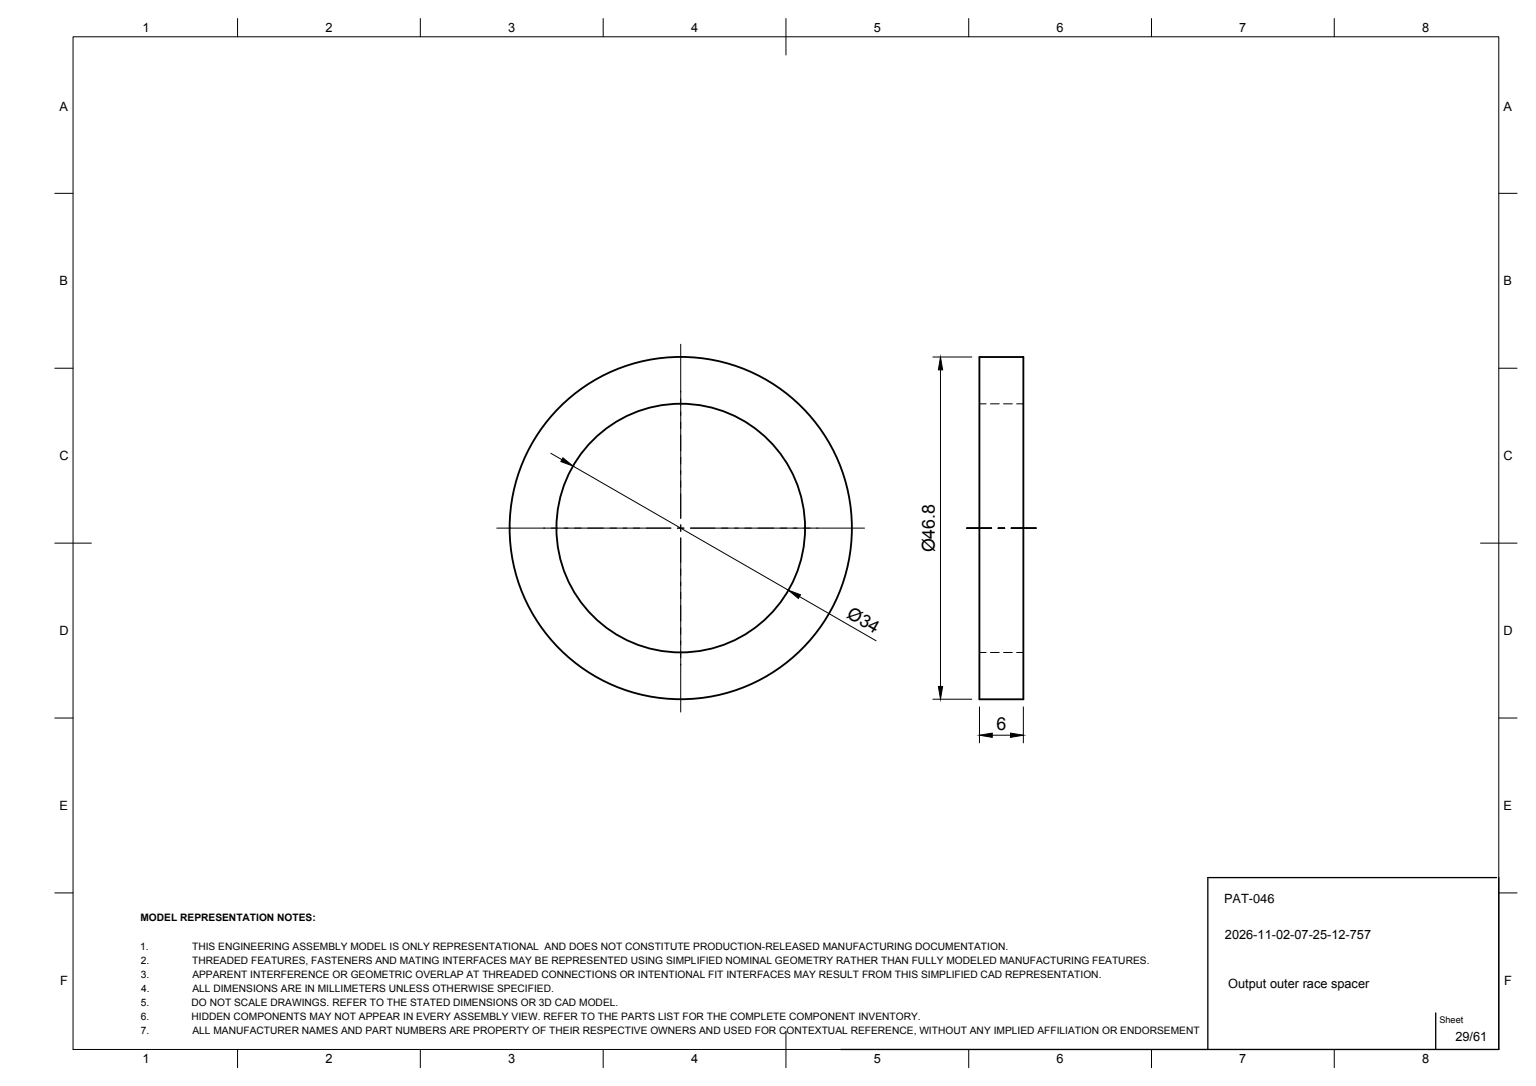
ISO-10303-21;
HEADER;
/* Generated by software containing ST-Developer
 * from STEP Tools, Inc. (www.steptools.com) 
 */

FILE_DESCRIPTION(
/* description */ ('Gear mesh backlash fixture'),
/* implementation_level */ '2;1');

FILE_NAME(
/* name */ 'Output outer race spacer.step',
/* time_stamp */ '2026-10-28T03:26:00-07:00',
/* author */ (''),
/* organization */ (''),
/* preprocessor_version */ 'ST-DEVELOPER v20.2',
/* originating_system */ 'Autodesk Translation Framework v15.17.0.0',
/* authorisation */ '');

FILE_SCHEMA (('AUTOMOTIVE_DESIGN { 1 0 10303 214 3 1 1 }'));
ENDSEC;

DATA;
#10=MECHANICAL_DESIGN_GEOMETRIC_PRESENTATION_REPRESENTATION('',(#1044),#57900);
#937=SHAPE_REPRESENTATION_RELATIONSHIP('SRR','None',#58134,#987);
#987=ADVANCED_BREP_SHAPE_REPRESENTATION('',(#1108),#57867);
#1044=STYLED_ITEM('',(#58465),#1108);
#1108=MANIFOLD_SOLID_BREP('Body1',#13605);
#1264=FACE_BOUND('',#2851,.T.);
#1265=FACE_BOUND('',#2853,.T.);
#1470=PLANE('',#14778);
#1471=PLANE('',#14779);
#1962=FACE_OUTER_BOUND('',#2848,.T.);
#1963=FACE_OUTER_BOUND('',#2849,.T.);
#1964=FACE_OUTER_BOUND('',#2850,.T.);
#1965=FACE_OUTER_BOUND('',#2852,.T.);
#2848=EDGE_LOOP('',(#10077,#10078,#10079,#10080));
#2849=EDGE_LOOP('',(#10081,#10082,#10083,#10084));
#2850=EDGE_LOOP('',(#10085));
#2851=EDGE_LOOP('',(#10086));
#2852=EDGE_LOOP('',(#10087));
#2853=EDGE_LOOP('',(#10088));
#3707=LINE('',#20994,#4596);
#3708=LINE('',#21000,#4597);
#4596=VECTOR('',#17032,1.7);
#4597=VECTOR('',#17039,2.34);
#5467=CIRCLE('',#14773,1.7);
#5468=CIRCLE('',#14774,1.7);
#5469=CIRCLE('',#14776,2.34);
#5470=CIRCLE('',#14777,2.34);
#6183=VERTEX_POINT('',#20991);
#6184=VERTEX_POINT('',#20993);
#6185=VERTEX_POINT('',#20997);
#6186=VERTEX_POINT('',#20999);
#7625=EDGE_CURVE('',#6183,#6183,#5467,.T.);
#7626=EDGE_CURVE('',#6183,#6184,#3707,.T.);
#7627=EDGE_CURVE('',#6184,#6184,#5468,.T.);
#7628=EDGE_CURVE('',#6185,#6185,#5469,.T.);
#7629=EDGE_CURVE('',#6185,#6186,#3708,.T.);
#7630=EDGE_CURVE('',#6186,#6186,#5470,.T.);
#10077=ORIENTED_EDGE('',*,*,#7625,.F.);
#10078=ORIENTED_EDGE('',*,*,#7626,.T.);
#10079=ORIENTED_EDGE('',*,*,#7627,.T.);
#10080=ORIENTED_EDGE('',*,*,#7626,.F.);
#10081=ORIENTED_EDGE('',*,*,#7628,.F.);
#10082=ORIENTED_EDGE('',*,*,#7629,.T.);
#10083=ORIENTED_EDGE('',*,*,#7630,.T.);
#10084=ORIENTED_EDGE('',*,*,#7629,.F.);
#10085=ORIENTED_EDGE('',*,*,#7628,.T.);
#10086=ORIENTED_EDGE('',*,*,#7625,.T.);
#10087=ORIENTED_EDGE('',*,*,#7630,.F.);
#10088=ORIENTED_EDGE('',*,*,#7627,.F.);
#12689=CYLINDRICAL_SURFACE('',#14772,1.7);
#12690=CYLINDRICAL_SURFACE('',#14775,2.34);
#13079=ADVANCED_FACE('',(#1962),#12689,.F.);
#13080=ADVANCED_FACE('',(#1963),#12690,.T.);
#13081=ADVANCED_FACE('',(#1964,#1264),#1470,.T.);
#13082=ADVANCED_FACE('',(#1965,#1265),#1471,.F.);
#13605=CLOSED_SHELL('',(#13079,#13080,#13081,#13082));
#14771=AXIS2_PLACEMENT_3D('',#20989,#17026,#17027);
#14772=AXIS2_PLACEMENT_3D('',#20990,#17028,#17029);
#14773=AXIS2_PLACEMENT_3D('',#20992,#17030,#17031);
#14774=AXIS2_PLACEMENT_3D('',#20995,#17033,#17034);
#14775=AXIS2_PLACEMENT_3D('',#20996,#17035,#17036);
#14776=AXIS2_PLACEMENT_3D('',#20998,#17037,#17038);
#14777=AXIS2_PLACEMENT_3D('',#21001,#17040,#17041);
#14778=AXIS2_PLACEMENT_3D('',#21002,#17042,#17043);
#14779=AXIS2_PLACEMENT_3D('',#21003,#17044,#17045);
#17026=DIRECTION('axis',(0.,0.,1.));
#17027=DIRECTION('refdir',(1.,0.,0.));
#17028=DIRECTION('center_axis',(0.,0.,1.));
#17029=DIRECTION('ref_axis',(1.,0.,0.));
#17030=DIRECTION('center_axis',(0.,0.,-1.));
#17031=DIRECTION('ref_axis',(1.,0.,0.));
#17032=DIRECTION('',(0.,0.,-1.));
#17033=DIRECTION('center_axis',(0.,0.,-1.));
#17034=DIRECTION('ref_axis',(1.,0.,0.));
#17035=DIRECTION('center_axis',(0.,0.,1.));
#17036=DIRECTION('ref_axis',(1.,0.,0.));
#17037=DIRECTION('center_axis',(0.,0.,1.));
#17038=DIRECTION('ref_axis',(1.,0.,0.));
#17039=DIRECTION('',(0.,0.,-1.));
#17040=DIRECTION('center_axis',(0.,0.,1.));
#17041=DIRECTION('ref_axis',(1.,0.,0.));
#17042=DIRECTION('center_axis',(0.,0.,1.));
#17043=DIRECTION('ref_axis',(1.,0.,0.));
#17044=DIRECTION('center_axis',(0.,0.,1.));
#17045=DIRECTION('ref_axis',(1.,0.,0.));
#20989=CARTESIAN_POINT('',(0.,0.,0.));
#20990=CARTESIAN_POINT('Origin',(6.,0.,7.2));
#20991=CARTESIAN_POINT('',(4.3,-2.0818995585505E-16,7.8));
#20992=CARTESIAN_POINT('Origin',(6.,0.,7.8));
#20993=CARTESIAN_POINT('',(4.3,-2.0818995585505E-16,7.2));
#20994=CARTESIAN_POINT('',(4.3,-2.0818995585505E-16,7.2));
#20995=CARTESIAN_POINT('Origin',(6.,0.,7.2));
#20996=CARTESIAN_POINT('Origin',(6.,0.,7.2));
#20997=CARTESIAN_POINT('',(3.66,-2.86567351000481E-16,7.8));
#20998=CARTESIAN_POINT('Origin',(6.,0.,7.8));
#20999=CARTESIAN_POINT('',(3.66,-2.86567351000481E-16,7.2));
#21000=CARTESIAN_POINT('',(3.66,-2.86567351000481E-16,7.2));
#21001=CARTESIAN_POINT('Origin',(6.,0.,7.2));
#21002=CARTESIAN_POINT('Origin',(6.,0.,7.8));
#21003=CARTESIAN_POINT('Origin',(6.,0.,7.2));
#57808=UNCERTAINTY_MEASURE_WITH_UNIT(LENGTH_MEASURE(0.001),#57901,
'DISTANCE_ACCURACY_VALUE',
'Maximum model space distance between geometric entities at asserted c
onnectivities');
#57841=UNCERTAINTY_MEASURE_WITH_UNIT(LENGTH_MEASURE(0.001),#57901,
'DISTANCE_ACCURACY_VALUE',
'Maximum model space distance between geometric entities at asserted c
onnectivities');
#57867=(
GEOMETRIC_REPRESENTATION_CONTEXT(3)
GLOBAL_UNCERTAINTY_ASSIGNED_CONTEXT((#57808))
GLOBAL_UNIT_ASSIGNED_CONTEXT((#57901,#57903,#57904))
REPRESENTATION_CONTEXT('','3D')
);
#57900=(
GEOMETRIC_REPRESENTATION_CONTEXT(3)
GLOBAL_UNCERTAINTY_ASSIGNED_CONTEXT((#57841))
GLOBAL_UNIT_ASSIGNED_CONTEXT((#57901,#57903,#57904))
REPRESENTATION_CONTEXT('','3D')
);
#57901=(
LENGTH_UNIT()
NAMED_UNIT(*)
SI_UNIT(.CENTI.,.METRE.)
);
#57903=(
NAMED_UNIT(*)
PLANE_ANGLE_UNIT()
SI_UNIT($,.RADIAN.)
);
#57904=(
NAMED_UNIT(*)
SI_UNIT($,.STERADIAN.)
SOLID_ANGLE_UNIT()
);
#57930=SHAPE_DEFINITION_REPRESENTATION(#57993,#58134);
#57993=PRODUCT_DEFINITION_SHAPE('',$,#58193);
#58134=SHAPE_REPRESENTATION('',(#14771),#57867);
#58167=PRODUCT_DEFINITION_CONTEXT('part definition',#58343,'design');
#58193=PRODUCT_DEFINITION('Output outer race spacer',
'Output outer race spacer',#58251,#58167);
#58251=PRODUCT_DEFINITION_FORMATION('',$,#58370);
#58343=APPLICATION_CONTEXT(
'Core Data for Automotive Mechanical Design Process');
#58344=PRODUCT_CONTEXT('part definition',#58343,'mechanical');
#58370=PRODUCT('Output outer race spacer','Output outer race spacer',
'Output outer race spacer',(#58344));
#58459=COLOUR_RGB('Grey',0.48,0.52,0.57);
#58460=FILL_AREA_STYLE_COLOUR('',#58459);
#58461=FILL_AREA_STYLE('',(#58460));
#58462=SURFACE_STYLE_FILL_AREA(#58461);
#58463=SURFACE_SIDE_STYLE('',(#58462));
#58464=SURFACE_STYLE_USAGE(.BOTH.,#58463);
#58465=PRESENTATION_STYLE_ASSIGNMENT((#58464));
ENDSEC;
END-ISO-10303-21;
